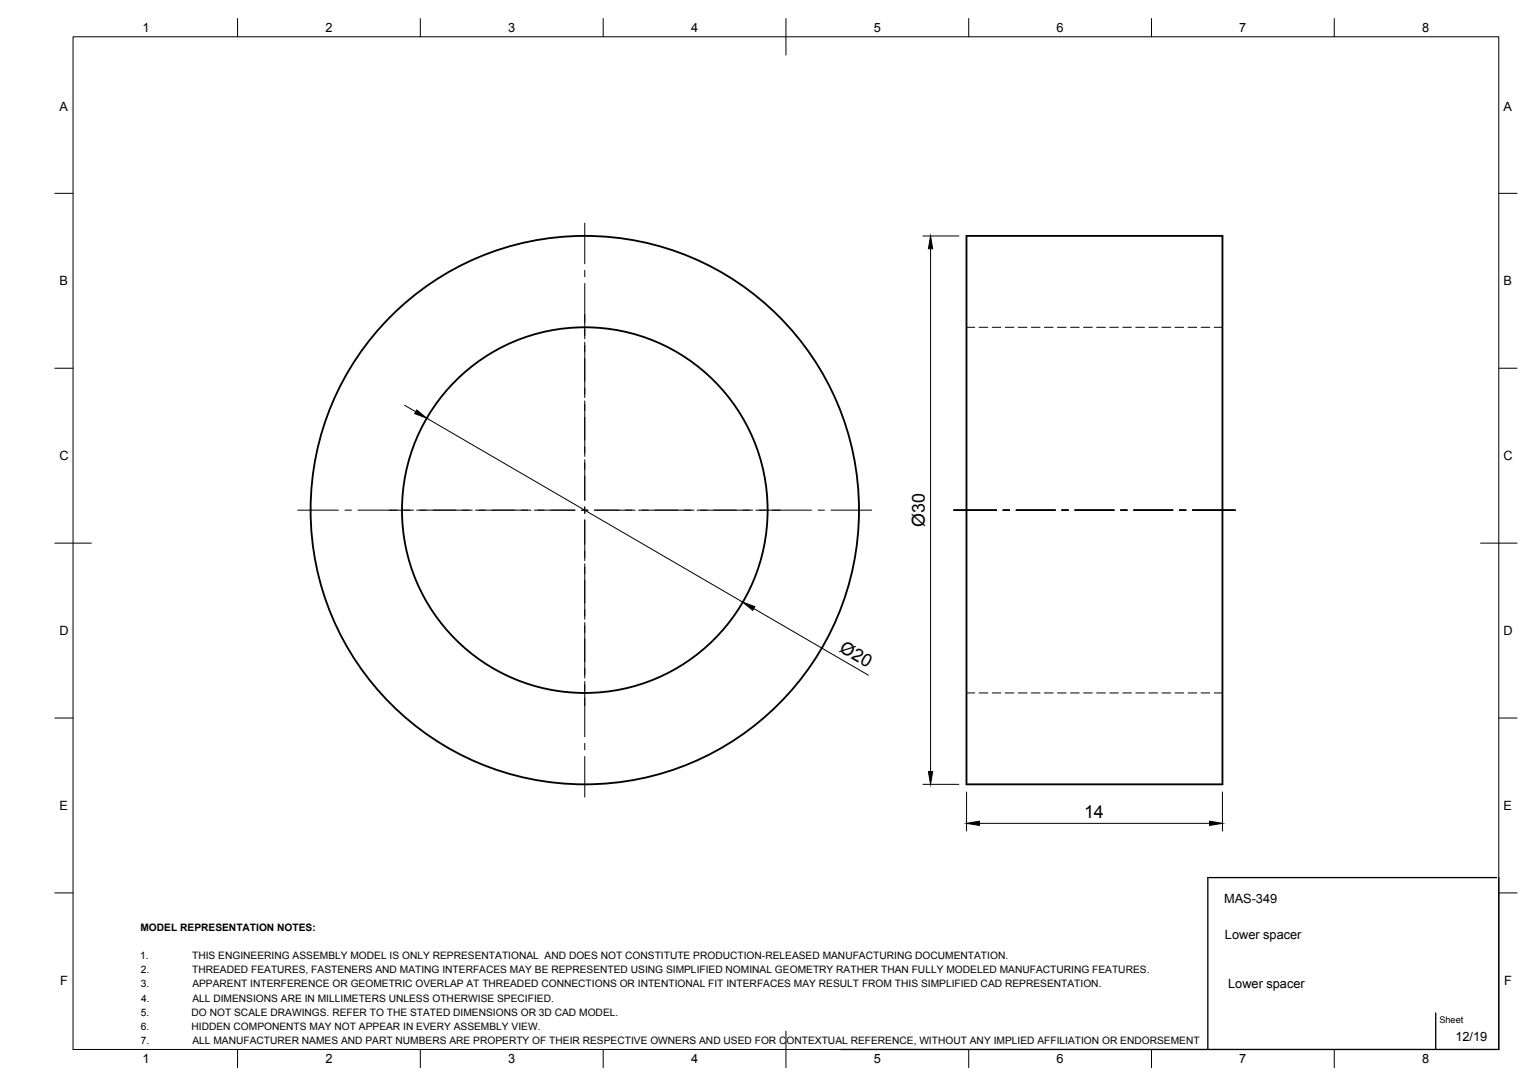
ISO-10303-21;
HEADER;
/* Generated by software containing ST-Developer
 * from STEP Tools, Inc. (www.steptools.com) 
 */

FILE_DESCRIPTION(
/* description */ ('Independent two-stage semi-open centrifugal-pump CAD. Shared impeller
s, open-machinable return casings, removable diaphragms, bronze wear/j
ournal rings, volume-preserving seal instances, retained keyed shaft, 
opposed mechanical face rings and partly threaded tie hardware. Native
 shaft rotation. Geometric topology/clearance only; flow/head/efficien
cy, pressure, cavitation, balance, preload, face loading and secondary
 seal fits/bonds, material/thermal/tolerance selection and life unassi
gned. External drive, coupling, anchors and piping bolts omitted.'),
/* implementation_level */ '2;1');

FILE_NAME(
/* name */ 'Lower spacer.step',
/* time_stamp */ '2026-11-08T18:06:32-08:00',
/* author */ (''),
/* organization */ (''),
/* preprocessor_version */ 'ST-DEVELOPER v20.2',
/* originating_system */ 'Autodesk Translation Framework v15.17.0.0',
/* authorisation */ '');

FILE_SCHEMA (('AUTOMOTIVE_DESIGN { 1 0 10303 214 3 1 1 }'));
ENDSEC;

DATA;
#10=MECHANICAL_DESIGN_GEOMETRIC_PRESENTATION_REPRESENTATION('',(#401),#16687);
#363=SHAPE_REPRESENTATION_RELATIONSHIP('SRR','None',#16772,#382);
#382=ADVANCED_BREP_SHAPE_REPRESENTATION('',(#420),#16676);
#401=STYLED_ITEM('',(#16874),#420);
#420=MANIFOLD_SOLID_BREP('Body1',#6120);
#535=FACE_BOUND('',#1412,.T.);
#536=FACE_BOUND('',#1414,.T.);
#651=PLANE('',#6831);
#652=PLANE('',#6832);
#958=FACE_OUTER_BOUND('',#1409,.T.);
#959=FACE_OUTER_BOUND('',#1410,.T.);
#960=FACE_OUTER_BOUND('',#1411,.T.);
#961=FACE_OUTER_BOUND('',#1413,.T.);
#1409=EDGE_LOOP('',(#5257,#5258,#5259,#5260));
#1410=EDGE_LOOP('',(#5261,#5262,#5263,#5264));
#1411=EDGE_LOOP('',(#5265));
#1412=EDGE_LOOP('',(#5266));
#1413=EDGE_LOOP('',(#5267));
#1414=EDGE_LOOP('',(#5268));
#1804=LINE('',#15105,#2173);
#1805=LINE('',#15111,#2174);
#2173=VECTOR('',#8262,1.);
#2174=VECTOR('',#8269,1.5);
#2450=CIRCLE('',#6826,1.);
#2451=CIRCLE('',#6827,1.);
#2452=CIRCLE('',#6829,1.5);
#2453=CIRCLE('',#6830,1.5);
#2953=VERTEX_POINT('',#15102);
#2954=VERTEX_POINT('',#15104);
#2955=VERTEX_POINT('',#15108);
#2956=VERTEX_POINT('',#15110);
#3738=EDGE_CURVE('',#2953,#2953,#2450,.T.);
#3739=EDGE_CURVE('',#2953,#2954,#1804,.T.);
#3740=EDGE_CURVE('',#2954,#2954,#2451,.T.);
#3741=EDGE_CURVE('',#2955,#2955,#2452,.T.);
#3742=EDGE_CURVE('',#2955,#2956,#1805,.T.);
#3743=EDGE_CURVE('',#2956,#2956,#2453,.T.);
#5257=ORIENTED_EDGE('',*,*,#3738,.F.);
#5258=ORIENTED_EDGE('',*,*,#3739,.T.);
#5259=ORIENTED_EDGE('',*,*,#3740,.T.);
#5260=ORIENTED_EDGE('',*,*,#3739,.F.);
#5261=ORIENTED_EDGE('',*,*,#3741,.F.);
#5262=ORIENTED_EDGE('',*,*,#3742,.T.);
#5263=ORIENTED_EDGE('',*,*,#3743,.T.);
#5264=ORIENTED_EDGE('',*,*,#3742,.F.);
#5265=ORIENTED_EDGE('',*,*,#3741,.T.);
#5266=ORIENTED_EDGE('',*,*,#3738,.T.);
#5267=ORIENTED_EDGE('',*,*,#3743,.F.);
#5268=ORIENTED_EDGE('',*,*,#3740,.F.);
#5728=CYLINDRICAL_SURFACE('',#6825,1.);
#5729=CYLINDRICAL_SURFACE('',#6828,1.5);
#6037=ADVANCED_FACE('',(#958),#5728,.F.);
#6038=ADVANCED_FACE('',(#959),#5729,.T.);
#6039=ADVANCED_FACE('',(#960,#535),#651,.T.);
#6040=ADVANCED_FACE('',(#961,#536),#652,.F.);
#6120=CLOSED_SHELL('',(#6037,#6038,#6039,#6040));
#6824=AXIS2_PLACEMENT_3D('',#15100,#8256,#8257);
#6825=AXIS2_PLACEMENT_3D('',#15101,#8258,#8259);
#6826=AXIS2_PLACEMENT_3D('',#15103,#8260,#8261);
#6827=AXIS2_PLACEMENT_3D('',#15106,#8263,#8264);
#6828=AXIS2_PLACEMENT_3D('',#15107,#8265,#8266);
#6829=AXIS2_PLACEMENT_3D('',#15109,#8267,#8268);
#6830=AXIS2_PLACEMENT_3D('',#15112,#8270,#8271);
#6831=AXIS2_PLACEMENT_3D('',#15113,#8272,#8273);
#6832=AXIS2_PLACEMENT_3D('',#15114,#8274,#8275);
#8256=DIRECTION('axis',(0.,0.,1.));
#8257=DIRECTION('refdir',(1.,0.,0.));
#8258=DIRECTION('center_axis',(0.,0.,1.));
#8259=DIRECTION('ref_axis',(1.,0.,0.));
#8260=DIRECTION('center_axis',(0.,0.,-1.));
#8261=DIRECTION('ref_axis',(1.,0.,0.));
#8262=DIRECTION('',(0.,0.,-1.));
#8263=DIRECTION('center_axis',(0.,0.,-1.));
#8264=DIRECTION('ref_axis',(1.,0.,0.));
#8265=DIRECTION('center_axis',(0.,0.,1.));
#8266=DIRECTION('ref_axis',(1.,0.,0.));
#8267=DIRECTION('center_axis',(0.,0.,1.));
#8268=DIRECTION('ref_axis',(1.,0.,0.));
#8269=DIRECTION('',(0.,0.,-1.));
#8270=DIRECTION('center_axis',(0.,0.,1.));
#8271=DIRECTION('ref_axis',(1.,0.,0.));
#8272=DIRECTION('center_axis',(0.,0.,1.));
#8273=DIRECTION('ref_axis',(1.,0.,0.));
#8274=DIRECTION('center_axis',(0.,0.,1.));
#8275=DIRECTION('ref_axis',(1.,0.,0.));
#15100=CARTESIAN_POINT('',(0.,0.,0.));
#15101=CARTESIAN_POINT('Origin',(0.,0.,0.4));
#15102=CARTESIAN_POINT('',(-1.,-1.22464679914735E-16,1.8));
#15103=CARTESIAN_POINT('Origin',(0.,0.,1.8));
#15104=CARTESIAN_POINT('',(-1.,-1.22464679914735E-16,0.4));
#15105=CARTESIAN_POINT('',(-1.,-1.22464679914735E-16,0.4));
#15106=CARTESIAN_POINT('Origin',(0.,0.,0.4));
#15107=CARTESIAN_POINT('Origin',(0.,0.,0.4));
#15108=CARTESIAN_POINT('',(-1.5,-1.83697019872103E-16,1.8));
#15109=CARTESIAN_POINT('Origin',(0.,0.,1.8));
#15110=CARTESIAN_POINT('',(-1.5,-1.83697019872103E-16,0.4));
#15111=CARTESIAN_POINT('',(-1.5,-1.83697019872103E-16,0.4));
#15112=CARTESIAN_POINT('Origin',(0.,0.,0.4));
#15113=CARTESIAN_POINT('Origin',(0.,0.,1.8));
#15114=CARTESIAN_POINT('Origin',(0.,0.,0.4));
#16655=UNCERTAINTY_MEASURE_WITH_UNIT(LENGTH_MEASURE(0.001),#16688,
'DISTANCE_ACCURACY_VALUE',
'Maximum model space distance between geometric entities at asserted c
onnectivities');
#16666=UNCERTAINTY_MEASURE_WITH_UNIT(LENGTH_MEASURE(0.001),#16688,
'DISTANCE_ACCURACY_VALUE',
'Maximum model space distance between geometric entities at asserted c
onnectivities');
#16676=(
GEOMETRIC_REPRESENTATION_CONTEXT(3)
GLOBAL_UNCERTAINTY_ASSIGNED_CONTEXT((#16655))
GLOBAL_UNIT_ASSIGNED_CONTEXT((#16688,#16690,#16691))
REPRESENTATION_CONTEXT('','3D')
);
#16687=(
GEOMETRIC_REPRESENTATION_CONTEXT(3)
GLOBAL_UNCERTAINTY_ASSIGNED_CONTEXT((#16666))
GLOBAL_UNIT_ASSIGNED_CONTEXT((#16688,#16690,#16691))
REPRESENTATION_CONTEXT('','3D')
);
#16688=(
LENGTH_UNIT()
NAMED_UNIT(*)
SI_UNIT(.CENTI.,.METRE.)
);
#16690=(
NAMED_UNIT(*)
PLANE_ANGLE_UNIT()
SI_UNIT($,.RADIAN.)
);
#16691=(
NAMED_UNIT(*)
SI_UNIT($,.STERADIAN.)
SOLID_ANGLE_UNIT()
);
#16701=SHAPE_DEFINITION_REPRESENTATION(#16721,#16772);
#16721=PRODUCT_DEFINITION_SHAPE('',$,#16793);
#16772=SHAPE_REPRESENTATION('',(#6824),#16676);
#16783=PRODUCT_DEFINITION_CONTEXT('part definition',#16845,'design');
#16793=PRODUCT_DEFINITION('Lower spacer','Lower spacer',#16813,#16783);
#16813=PRODUCT_DEFINITION_FORMATION('',$,#16856);
#16845=APPLICATION_CONTEXT(
'Core Data for Automotive Mechanical Design Process');
#16846=PRODUCT_CONTEXT('part definition',#16845,'mechanical');
#16856=PRODUCT('Lower spacer','Lower spacer',$,(#16846));
#16874=PRESENTATION_STYLE_ASSIGNMENT((#16889));
#16889=SURFACE_STYLE_USAGE(.BOTH.,#16904);
#16904=SURFACE_SIDE_STYLE('',(#16919));
#16919=SURFACE_STYLE_FILL_AREA(#16934);
#16934=FILL_AREA_STYLE('Spacer gray',(#16949));
#16949=FILL_AREA_STYLE_COLOUR('Spacer gray',#16964);
#16964=COLOUR_RGB('Spacer gray',0.576470588235294,0.615686274509804,0.666666666666667);
ENDSEC;
END-ISO-10303-21;
